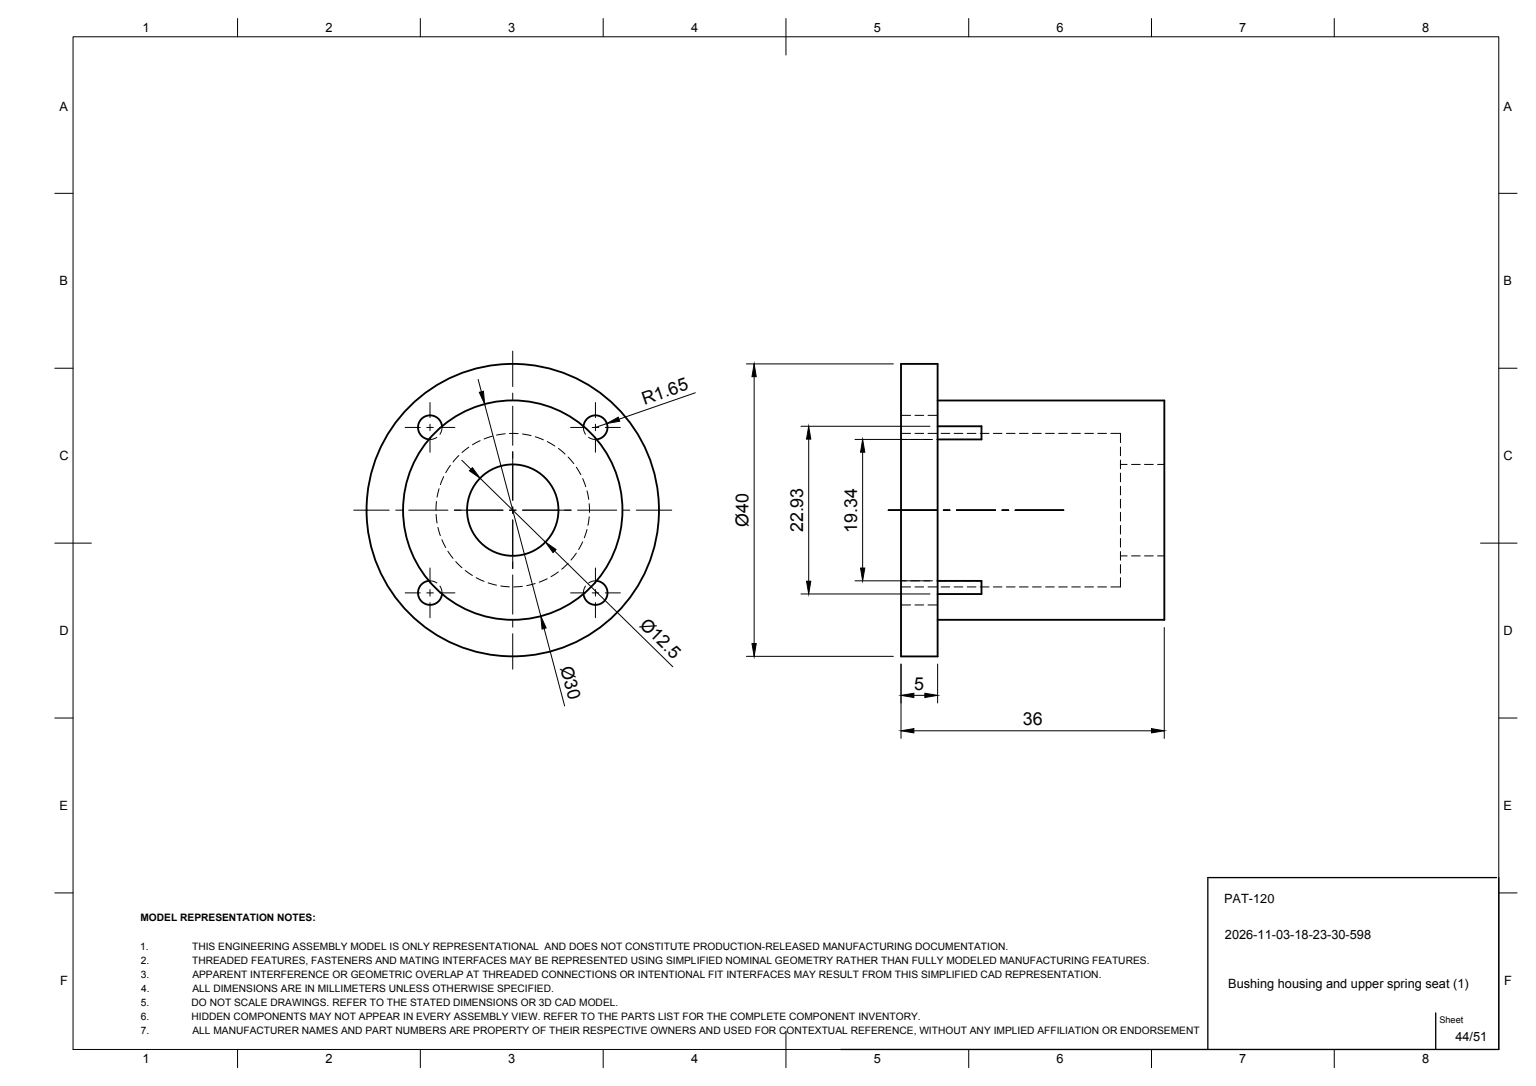
ISO-10303-21;
HEADER;
/* Generated by software containing ST-Developer
 * from STEP Tools, Inc. (www.steptools.com) 
 */

FILE_DESCRIPTION(
/* description */ ('Vibration shaker table dummy'),
/* implementation_level */ '2;1');

FILE_NAME(
/* name */ 'Bushing housing and upper spring seat (1).step',
/* time_stamp */ '2026-10-27T10:55:14-07:00',
/* author */ (''),
/* organization */ (''),
/* preprocessor_version */ 'ST-DEVELOPER v20.2',
/* originating_system */ 'Autodesk Translation Framework v15.17.0.0',
/* authorisation */ '');

FILE_SCHEMA (('AUTOMOTIVE_DESIGN { 1 0 10303 214 3 1 1 }'));
ENDSEC;

DATA;
#10=MECHANICAL_DESIGN_GEOMETRIC_PRESENTATION_REPRESENTATION('',(#725),#22394);
#633=SHAPE_REPRESENTATION_RELATIONSHIP('SRR','None',#22680,#679);
#679=ADVANCED_BREP_SHAPE_REPRESENTATION('',(#769),#22386);
#725=STYLED_ITEM('',(#22961),#769);
#769=MANIFOLD_SOLID_BREP('Body1',#9245);
#1015=FACE_BOUND('',#2489,.T.);
#1016=FACE_BOUND('',#2491,.T.);
#1017=FACE_BOUND('',#2495,.T.);
#1018=FACE_BOUND('',#2496,.T.);
#1019=FACE_BOUND('',#2497,.T.);
#1020=FACE_BOUND('',#2498,.T.);
#1021=FACE_BOUND('',#2499,.T.);
#1022=FACE_BOUND('',#2501,.T.);
#1286=PLANE('',#10567);
#1287=PLANE('',#10574);
#1288=PLANE('',#10581);
#1289=PLANE('',#10588);
#1290=PLANE('',#10605);
#1291=PLANE('',#10607);
#1292=PLANE('',#10613);
#1293=PLANE('',#10614);
#1740=FACE_OUTER_BOUND('',#2478,.T.);
#1741=FACE_OUTER_BOUND('',#2479,.T.);
#1742=FACE_OUTER_BOUND('',#2480,.T.);
#1743=FACE_OUTER_BOUND('',#2481,.T.);
#1744=FACE_OUTER_BOUND('',#2482,.T.);
#1745=FACE_OUTER_BOUND('',#2483,.T.);
#1746=FACE_OUTER_BOUND('',#2484,.T.);
#1747=FACE_OUTER_BOUND('',#2485,.T.);
#1748=FACE_OUTER_BOUND('',#2486,.T.);
#1749=FACE_OUTER_BOUND('',#2487,.T.);
#1750=FACE_OUTER_BOUND('',#2488,.T.);
#1751=FACE_OUTER_BOUND('',#2490,.T.);
#1752=FACE_OUTER_BOUND('',#2492,.T.);
#1753=FACE_OUTER_BOUND('',#2493,.T.);
#1754=FACE_OUTER_BOUND('',#2494,.T.);
#1755=FACE_OUTER_BOUND('',#2500,.T.);
#2478=EDGE_LOOP('',(#8022,#8023));
#2479=EDGE_LOOP('',(#8024,#8025,#8026,#8027,#8028,#8029,#8030,#8031));
#2480=EDGE_LOOP('',(#8032,#8033));
#2481=EDGE_LOOP('',(#8034,#8035,#8036,#8037,#8038,#8039,#8040,#8041));
#2482=EDGE_LOOP('',(#8042,#8043,#8044));
#2483=EDGE_LOOP('',(#8045,#8046,#8047,#8048,#8049,#8050,#8051,#8052));
#2484=EDGE_LOOP('',(#8053,#8054,#8055));
#2485=EDGE_LOOP('',(#8056,#8057,#8058,#8059,#8060,#8061,#8062,#8063));
#2486=EDGE_LOOP('',(#8064,#8065,#8066,#8067,#8068,#8069,#8070,#8071,#8072,
#8073,#8074,#8075,#8076,#8077,#8078,#8079,#8080,#8081,#8082,#8083));
#2487=EDGE_LOOP('',(#8084,#8085,#8086,#8087));
#2488=EDGE_LOOP('',(#8088));
#2489=EDGE_LOOP('',(#8089));
#2490=EDGE_LOOP('',(#8090));
#2491=EDGE_LOOP('',(#8091,#8092,#8093,#8094,#8095,#8096,#8097,#8098,#8099,
#8100,#8101));
#2492=EDGE_LOOP('',(#8102,#8103,#8104,#8105));
#2493=EDGE_LOOP('',(#8106,#8107,#8108,#8109));
#2494=EDGE_LOOP('',(#8110));
#2495=EDGE_LOOP('',(#8111));
#2496=EDGE_LOOP('',(#8112));
#2497=EDGE_LOOP('',(#8113));
#2498=EDGE_LOOP('',(#8114));
#2499=EDGE_LOOP('',(#8115));
#2500=EDGE_LOOP('',(#8116));
#2501=EDGE_LOOP('',(#8117));
#3137=LINE('',#21653,#3756);
#3138=LINE('',#21657,#3757);
#3139=LINE('',#21661,#3758);
#3140=LINE('',#21669,#3759);
#3141=LINE('',#21673,#3760);
#3142=LINE('',#21677,#3761);
#3143=LINE('',#21687,#3762);
#3144=LINE('',#21690,#3763);
#3145=LINE('',#21692,#3764);
#3146=LINE('',#21703,#3765);
#3147=LINE('',#21706,#3766);
#3148=LINE('',#21708,#3767);
#3149=LINE('',#21714,#3768);
#3150=LINE('',#21724,#3769);
#3151=LINE('',#21735,#3770);
#3152=LINE('',#21738,#3771);
#3756=VECTOR('',#13087,1.);
#3757=VECTOR('',#13090,0.165);
#3758=VECTOR('',#13095,1.);
#3759=VECTOR('',#13104,1.);
#3760=VECTOR('',#13107,0.165);
#3761=VECTOR('',#13112,1.);
#3762=VECTOR('',#13123,1.);
#3763=VECTOR('',#13126,1.);
#3764=VECTOR('',#13127,0.165);
#3765=VECTOR('',#13140,1.);
#3766=VECTOR('',#13143,1.);
#3767=VECTOR('',#13144,0.165);
#3768=VECTOR('',#13151,1.5);
#3769=VECTOR('',#13166,1.05);
#3770=VECTOR('',#13181,2.);
#3771=VECTOR('',#13184,0.625);
#4229=CIRCLE('',#10568,1.5);
#4230=CIRCLE('',#10569,0.165);
#4231=CIRCLE('',#10571,0.165);
#4232=CIRCLE('',#10572,0.165);
#4233=CIRCLE('',#10573,0.165);
#4234=CIRCLE('',#10575,1.5);
#4235=CIRCLE('',#10576,0.165);
#4236=CIRCLE('',#10578,0.165);
#4237=CIRCLE('',#10579,0.165);
#4238=CIRCLE('',#10580,0.165);
#4239=CIRCLE('',#10582,1.5);
#4240=CIRCLE('',#10583,0.165);
#4241=CIRCLE('',#10584,0.165);
#4242=CIRCLE('',#10586,0.165);
#4243=CIRCLE('',#10587,0.165);
#4244=CIRCLE('',#10589,1.5);
#4245=CIRCLE('',#10590,0.165);
#4246=CIRCLE('',#10591,0.165);
#4247=CIRCLE('',#10593,0.165);
#4248=CIRCLE('',#10594,0.165);
#4249=CIRCLE('',#10596,1.5);
#4250=CIRCLE('',#10597,1.5);
#4251=CIRCLE('',#10598,1.5);
#4252=CIRCLE('',#10599,1.5);
#4253=CIRCLE('',#10600,1.5);
#4254=CIRCLE('',#10601,1.5);
#4255=CIRCLE('',#10603,1.05);
#4256=CIRCLE('',#10604,1.05);
#4257=CIRCLE('',#10606,0.625);
#4258=CIRCLE('',#10608,2.);
#4259=CIRCLE('',#10610,2.);
#4260=CIRCLE('',#10612,0.625);
#4956=VERTEX_POINT('',#21647);
#4957=VERTEX_POINT('',#21648);
#4958=VERTEX_POINT('',#21652);
#4959=VERTEX_POINT('',#21654);
#4960=VERTEX_POINT('',#21656);
#4961=VERTEX_POINT('',#21659);
#4962=VERTEX_POINT('',#21663);
#4963=VERTEX_POINT('',#21664);
#4964=VERTEX_POINT('',#21668);
#4965=VERTEX_POINT('',#21670);
#4966=VERTEX_POINT('',#21672);
#4967=VERTEX_POINT('',#21675);
#4968=VERTEX_POINT('',#21679);
#4969=VERTEX_POINT('',#21680);
#4970=VERTEX_POINT('',#21682);
#4971=VERTEX_POINT('',#21686);
#4972=VERTEX_POINT('',#21688);
#4973=VERTEX_POINT('',#21691);
#4974=VERTEX_POINT('',#21695);
#4975=VERTEX_POINT('',#21696);
#4976=VERTEX_POINT('',#21698);
#4977=VERTEX_POINT('',#21702);
#4978=VERTEX_POINT('',#21704);
#4979=VERTEX_POINT('',#21707);
#4980=VERTEX_POINT('',#21711);
#4981=VERTEX_POINT('',#21713);
#4982=VERTEX_POINT('',#21721);
#4983=VERTEX_POINT('',#21723);
#4984=VERTEX_POINT('',#21727);
#4985=VERTEX_POINT('',#21730);
#4986=VERTEX_POINT('',#21733);
#4987=VERTEX_POINT('',#21737);
#6004=EDGE_CURVE('',#4956,#4957,#4229,.T.);
#6005=EDGE_CURVE('',#4956,#4957,#4230,.T.);
#6006=EDGE_CURVE('',#4958,#4956,#3137,.T.);
#6007=EDGE_CURVE('',#4959,#4958,#4231,.T.);
#6008=EDGE_CURVE('',#4959,#4960,#3138,.T.);
#6009=EDGE_CURVE('',#4960,#4960,#4232,.T.);
#6010=EDGE_CURVE('',#4961,#4959,#4233,.T.);
#6011=EDGE_CURVE('',#4957,#4961,#3139,.T.);
#6012=EDGE_CURVE('',#4962,#4963,#4234,.T.);
#6013=EDGE_CURVE('',#4962,#4963,#4235,.T.);
#6014=EDGE_CURVE('',#4964,#4962,#3140,.T.);
#6015=EDGE_CURVE('',#4965,#4964,#4236,.T.);
#6016=EDGE_CURVE('',#4965,#4966,#3141,.T.);
#6017=EDGE_CURVE('',#4966,#4966,#4237,.T.);
#6018=EDGE_CURVE('',#4967,#4965,#4238,.T.);
#6019=EDGE_CURVE('',#4963,#4967,#3142,.T.);
#6020=EDGE_CURVE('',#4968,#4969,#4239,.T.);
#6021=EDGE_CURVE('',#4968,#4970,#4240,.T.);
#6022=EDGE_CURVE('',#4970,#4969,#4241,.T.);
#6023=EDGE_CURVE('',#4971,#4968,#3143,.T.);
#6024=EDGE_CURVE('',#4972,#4971,#4242,.T.);
#6025=EDGE_CURVE('',#4969,#4972,#3144,.T.);
#6026=EDGE_CURVE('',#4970,#4973,#3145,.T.);
#6027=EDGE_CURVE('',#4973,#4973,#4243,.T.);
#6028=EDGE_CURVE('',#4974,#4975,#4244,.T.);
#6029=EDGE_CURVE('',#4974,#4976,#4245,.T.);
#6030=EDGE_CURVE('',#4976,#4975,#4246,.T.);
#6031=EDGE_CURVE('',#4977,#4974,#3146,.T.);
#6032=EDGE_CURVE('',#4978,#4977,#4247,.T.);
#6033=EDGE_CURVE('',#4975,#4978,#3147,.T.);
#6034=EDGE_CURVE('',#4976,#4979,#3148,.T.);
#6035=EDGE_CURVE('',#4979,#4979,#4248,.T.);
#6036=EDGE_CURVE('',#4961,#4980,#4249,.T.);
#6037=EDGE_CURVE('',#4980,#4981,#3149,.T.);
#6038=EDGE_CURVE('',#4981,#4981,#4250,.T.);
#6039=EDGE_CURVE('',#4980,#4964,#4251,.T.);
#6040=EDGE_CURVE('',#4967,#4971,#4252,.T.);
#6041=EDGE_CURVE('',#4972,#4977,#4253,.T.);
#6042=EDGE_CURVE('',#4978,#4958,#4254,.T.);
#6043=EDGE_CURVE('',#4982,#4982,#4255,.T.);
#6044=EDGE_CURVE('',#4982,#4983,#3150,.T.);
#6045=EDGE_CURVE('',#4983,#4983,#4256,.T.);
#6046=EDGE_CURVE('',#4984,#4984,#4257,.T.);
#6047=EDGE_CURVE('',#4985,#4985,#4258,.T.);
#6048=EDGE_CURVE('',#4986,#4986,#4259,.T.);
#6049=EDGE_CURVE('',#4986,#4985,#3151,.T.);
#6050=EDGE_CURVE('',#4984,#4987,#3152,.T.);
#6051=EDGE_CURVE('',#4987,#4987,#4260,.T.);
#8022=ORIENTED_EDGE('',*,*,#6004,.F.);
#8023=ORIENTED_EDGE('',*,*,#6005,.T.);
#8024=ORIENTED_EDGE('',*,*,#6006,.F.);
#8025=ORIENTED_EDGE('',*,*,#6007,.F.);
#8026=ORIENTED_EDGE('',*,*,#6008,.T.);
#8027=ORIENTED_EDGE('',*,*,#6009,.F.);
#8028=ORIENTED_EDGE('',*,*,#6008,.F.);
#8029=ORIENTED_EDGE('',*,*,#6010,.F.);
#8030=ORIENTED_EDGE('',*,*,#6011,.F.);
#8031=ORIENTED_EDGE('',*,*,#6005,.F.);
#8032=ORIENTED_EDGE('',*,*,#6012,.F.);
#8033=ORIENTED_EDGE('',*,*,#6013,.T.);
#8034=ORIENTED_EDGE('',*,*,#6014,.F.);
#8035=ORIENTED_EDGE('',*,*,#6015,.F.);
#8036=ORIENTED_EDGE('',*,*,#6016,.T.);
#8037=ORIENTED_EDGE('',*,*,#6017,.F.);
#8038=ORIENTED_EDGE('',*,*,#6016,.F.);
#8039=ORIENTED_EDGE('',*,*,#6018,.F.);
#8040=ORIENTED_EDGE('',*,*,#6019,.F.);
#8041=ORIENTED_EDGE('',*,*,#6013,.F.);
#8042=ORIENTED_EDGE('',*,*,#6020,.F.);
#8043=ORIENTED_EDGE('',*,*,#6021,.T.);
#8044=ORIENTED_EDGE('',*,*,#6022,.T.);
#8045=ORIENTED_EDGE('',*,*,#6023,.F.);
#8046=ORIENTED_EDGE('',*,*,#6024,.F.);
#8047=ORIENTED_EDGE('',*,*,#6025,.F.);
#8048=ORIENTED_EDGE('',*,*,#6022,.F.);
#8049=ORIENTED_EDGE('',*,*,#6026,.T.);
#8050=ORIENTED_EDGE('',*,*,#6027,.F.);
#8051=ORIENTED_EDGE('',*,*,#6026,.F.);
#8052=ORIENTED_EDGE('',*,*,#6021,.F.);
#8053=ORIENTED_EDGE('',*,*,#6028,.F.);
#8054=ORIENTED_EDGE('',*,*,#6029,.T.);
#8055=ORIENTED_EDGE('',*,*,#6030,.T.);
#8056=ORIENTED_EDGE('',*,*,#6031,.F.);
#8057=ORIENTED_EDGE('',*,*,#6032,.F.);
#8058=ORIENTED_EDGE('',*,*,#6033,.F.);
#8059=ORIENTED_EDGE('',*,*,#6030,.F.);
#8060=ORIENTED_EDGE('',*,*,#6034,.T.);
#8061=ORIENTED_EDGE('',*,*,#6035,.F.);
#8062=ORIENTED_EDGE('',*,*,#6034,.F.);
#8063=ORIENTED_EDGE('',*,*,#6029,.F.);
#8064=ORIENTED_EDGE('',*,*,#6006,.T.);
#8065=ORIENTED_EDGE('',*,*,#6004,.T.);
#8066=ORIENTED_EDGE('',*,*,#6011,.T.);
#8067=ORIENTED_EDGE('',*,*,#6036,.T.);
#8068=ORIENTED_EDGE('',*,*,#6037,.T.);
#8069=ORIENTED_EDGE('',*,*,#6038,.T.);
#8070=ORIENTED_EDGE('',*,*,#6037,.F.);
#8071=ORIENTED_EDGE('',*,*,#6039,.T.);
#8072=ORIENTED_EDGE('',*,*,#6014,.T.);
#8073=ORIENTED_EDGE('',*,*,#6012,.T.);
#8074=ORIENTED_EDGE('',*,*,#6019,.T.);
#8075=ORIENTED_EDGE('',*,*,#6040,.T.);
#8076=ORIENTED_EDGE('',*,*,#6023,.T.);
#8077=ORIENTED_EDGE('',*,*,#6020,.T.);
#8078=ORIENTED_EDGE('',*,*,#6025,.T.);
#8079=ORIENTED_EDGE('',*,*,#6041,.T.);
#8080=ORIENTED_EDGE('',*,*,#6031,.T.);
#8081=ORIENTED_EDGE('',*,*,#6028,.T.);
#8082=ORIENTED_EDGE('',*,*,#6033,.T.);
#8083=ORIENTED_EDGE('',*,*,#6042,.T.);
#8084=ORIENTED_EDGE('',*,*,#6043,.F.);
#8085=ORIENTED_EDGE('',*,*,#6044,.T.);
#8086=ORIENTED_EDGE('',*,*,#6045,.F.);
#8087=ORIENTED_EDGE('',*,*,#6044,.F.);
#8088=ORIENTED_EDGE('',*,*,#6043,.T.);
#8089=ORIENTED_EDGE('',*,*,#6046,.F.);
#8090=ORIENTED_EDGE('',*,*,#6047,.F.);
#8091=ORIENTED_EDGE('',*,*,#6010,.T.);
#8092=ORIENTED_EDGE('',*,*,#6007,.T.);
#8093=ORIENTED_EDGE('',*,*,#6042,.F.);
#8094=ORIENTED_EDGE('',*,*,#6032,.T.);
#8095=ORIENTED_EDGE('',*,*,#6041,.F.);
#8096=ORIENTED_EDGE('',*,*,#6024,.T.);
#8097=ORIENTED_EDGE('',*,*,#6040,.F.);
#8098=ORIENTED_EDGE('',*,*,#6018,.T.);
#8099=ORIENTED_EDGE('',*,*,#6015,.T.);
#8100=ORIENTED_EDGE('',*,*,#6039,.F.);
#8101=ORIENTED_EDGE('',*,*,#6036,.F.);
#8102=ORIENTED_EDGE('',*,*,#6048,.F.);
#8103=ORIENTED_EDGE('',*,*,#6049,.T.);
#8104=ORIENTED_EDGE('',*,*,#6047,.T.);
#8105=ORIENTED_EDGE('',*,*,#6049,.F.);
#8106=ORIENTED_EDGE('',*,*,#6046,.T.);
#8107=ORIENTED_EDGE('',*,*,#6050,.T.);
#8108=ORIENTED_EDGE('',*,*,#6051,.T.);
#8109=ORIENTED_EDGE('',*,*,#6050,.F.);
#8110=ORIENTED_EDGE('',*,*,#6048,.T.);
#8111=ORIENTED_EDGE('',*,*,#6045,.T.);
#8112=ORIENTED_EDGE('',*,*,#6035,.T.);
#8113=ORIENTED_EDGE('',*,*,#6027,.T.);
#8114=ORIENTED_EDGE('',*,*,#6017,.T.);
#8115=ORIENTED_EDGE('',*,*,#6009,.T.);
#8116=ORIENTED_EDGE('',*,*,#6038,.F.);
#8117=ORIENTED_EDGE('',*,*,#6051,.F.);
#8666=CYLINDRICAL_SURFACE('',#10570,0.165);
#8667=CYLINDRICAL_SURFACE('',#10577,0.165);
#8668=CYLINDRICAL_SURFACE('',#10585,0.165);
#8669=CYLINDRICAL_SURFACE('',#10592,0.165);
#8670=CYLINDRICAL_SURFACE('',#10595,1.5);
#8671=CYLINDRICAL_SURFACE('',#10602,1.05);
#8672=CYLINDRICAL_SURFACE('',#10609,2.);
#8673=CYLINDRICAL_SURFACE('',#10611,0.625);
#9105=ADVANCED_FACE('',(#1740),#1286,.T.);
#9106=ADVANCED_FACE('',(#1741),#8666,.F.);
#9107=ADVANCED_FACE('',(#1742),#1287,.T.);
#9108=ADVANCED_FACE('',(#1743),#8667,.F.);
#9109=ADVANCED_FACE('',(#1744),#1288,.T.);
#9110=ADVANCED_FACE('',(#1745),#8668,.F.);
#9111=ADVANCED_FACE('',(#1746),#1289,.T.);
#9112=ADVANCED_FACE('',(#1747),#8669,.F.);
#9113=ADVANCED_FACE('',(#1748),#8670,.T.);
#9114=ADVANCED_FACE('',(#1749),#8671,.F.);
#9115=ADVANCED_FACE('',(#1750,#1015),#1290,.T.);
#9116=ADVANCED_FACE('',(#1751,#1016),#1291,.F.);
#9117=ADVANCED_FACE('',(#1752),#8672,.T.);
#9118=ADVANCED_FACE('',(#1753),#8673,.F.);
#9119=ADVANCED_FACE('',(#1754,#1017,#1018,#1019,#1020,#1021),#1292,.T.);
#9120=ADVANCED_FACE('',(#1755,#1022),#1293,.F.);
#9245=CLOSED_SHELL('',(#9105,#9106,#9107,#9108,#9109,#9110,#9111,#9112,
#9113,#9114,#9115,#9116,#9117,#9118,#9119,#9120));
#10566=AXIS2_PLACEMENT_3D('',#21645,#13077,#13078);
#10567=AXIS2_PLACEMENT_3D('',#21646,#13079,#13080);
#10568=AXIS2_PLACEMENT_3D('',#21649,#13081,#13082);
#10569=AXIS2_PLACEMENT_3D('',#21650,#13083,#13084);
#10570=AXIS2_PLACEMENT_3D('',#21651,#13085,#13086);
#10571=AXIS2_PLACEMENT_3D('',#21655,#13088,#13089);
#10572=AXIS2_PLACEMENT_3D('',#21658,#13091,#13092);
#10573=AXIS2_PLACEMENT_3D('',#21660,#13093,#13094);
#10574=AXIS2_PLACEMENT_3D('',#21662,#13096,#13097);
#10575=AXIS2_PLACEMENT_3D('',#21665,#13098,#13099);
#10576=AXIS2_PLACEMENT_3D('',#21666,#13100,#13101);
#10577=AXIS2_PLACEMENT_3D('',#21667,#13102,#13103);
#10578=AXIS2_PLACEMENT_3D('',#21671,#13105,#13106);
#10579=AXIS2_PLACEMENT_3D('',#21674,#13108,#13109);
#10580=AXIS2_PLACEMENT_3D('',#21676,#13110,#13111);
#10581=AXIS2_PLACEMENT_3D('',#21678,#13113,#13114);
#10582=AXIS2_PLACEMENT_3D('',#21681,#13115,#13116);
#10583=AXIS2_PLACEMENT_3D('',#21683,#13117,#13118);
#10584=AXIS2_PLACEMENT_3D('',#21684,#13119,#13120);
#10585=AXIS2_PLACEMENT_3D('',#21685,#13121,#13122);
#10586=AXIS2_PLACEMENT_3D('',#21689,#13124,#13125);
#10587=AXIS2_PLACEMENT_3D('',#21693,#13128,#13129);
#10588=AXIS2_PLACEMENT_3D('',#21694,#13130,#13131);
#10589=AXIS2_PLACEMENT_3D('',#21697,#13132,#13133);
#10590=AXIS2_PLACEMENT_3D('',#21699,#13134,#13135);
#10591=AXIS2_PLACEMENT_3D('',#21700,#13136,#13137);
#10592=AXIS2_PLACEMENT_3D('',#21701,#13138,#13139);
#10593=AXIS2_PLACEMENT_3D('',#21705,#13141,#13142);
#10594=AXIS2_PLACEMENT_3D('',#21709,#13145,#13146);
#10595=AXIS2_PLACEMENT_3D('',#21710,#13147,#13148);
#10596=AXIS2_PLACEMENT_3D('',#21712,#13149,#13150);
#10597=AXIS2_PLACEMENT_3D('',#21715,#13152,#13153);
#10598=AXIS2_PLACEMENT_3D('',#21716,#13154,#13155);
#10599=AXIS2_PLACEMENT_3D('',#21717,#13156,#13157);
#10600=AXIS2_PLACEMENT_3D('',#21718,#13158,#13159);
#10601=AXIS2_PLACEMENT_3D('',#21719,#13160,#13161);
#10602=AXIS2_PLACEMENT_3D('',#21720,#13162,#13163);
#10603=AXIS2_PLACEMENT_3D('',#21722,#13164,#13165);
#10604=AXIS2_PLACEMENT_3D('',#21725,#13167,#13168);
#10605=AXIS2_PLACEMENT_3D('',#21726,#13169,#13170);
#10606=AXIS2_PLACEMENT_3D('',#21728,#13171,#13172);
#10607=AXIS2_PLACEMENT_3D('',#21729,#13173,#13174);
#10608=AXIS2_PLACEMENT_3D('',#21731,#13175,#13176);
#10609=AXIS2_PLACEMENT_3D('',#21732,#13177,#13178);
#10610=AXIS2_PLACEMENT_3D('',#21734,#13179,#13180);
#10611=AXIS2_PLACEMENT_3D('',#21736,#13182,#13183);
#10612=AXIS2_PLACEMENT_3D('',#21739,#13185,#13186);
#10613=AXIS2_PLACEMENT_3D('',#21740,#13187,#13188);
#10614=AXIS2_PLACEMENT_3D('',#21741,#13189,#13190);
#13077=DIRECTION('axis',(0.,0.,1.));
#13078=DIRECTION('refdir',(1.,0.,0.));
#13079=DIRECTION('center_axis',(0.,0.,1.));
#13080=DIRECTION('ref_axis',(1.,0.,0.));
#13081=DIRECTION('center_axis',(0.,0.,-1.));
#13082=DIRECTION('ref_axis',(1.,0.,0.));
#13083=DIRECTION('center_axis',(0.,0.,1.));
#13084=DIRECTION('ref_axis',(1.,0.,0.));
#13085=DIRECTION('center_axis',(0.,0.,1.));
#13086=DIRECTION('ref_axis',(1.,0.,0.));
#13087=DIRECTION('',(0.,0.,-1.));
#13088=DIRECTION('center_axis',(0.,0.,1.));
#13089=DIRECTION('ref_axis',(1.,0.,0.));
#13090=DIRECTION('',(0.,0.,1.));
#13091=DIRECTION('center_axis',(0.,0.,-1.));
#13092=DIRECTION('ref_axis',(1.,0.,0.));
#13093=DIRECTION('center_axis',(0.,0.,1.));
#13094=DIRECTION('ref_axis',(1.,0.,0.));
#13095=DIRECTION('',(0.,0.,1.));
#13096=DIRECTION('center_axis',(0.,0.,1.));
#13097=DIRECTION('ref_axis',(1.,0.,0.));
#13098=DIRECTION('center_axis',(0.,0.,-1.));
#13099=DIRECTION('ref_axis',(1.,0.,0.));
#13100=DIRECTION('center_axis',(0.,0.,1.));
#13101=DIRECTION('ref_axis',(1.,0.,0.));
#13102=DIRECTION('center_axis',(0.,0.,1.));
#13103=DIRECTION('ref_axis',(1.,0.,0.));
#13104=DIRECTION('',(0.,0.,-1.));
#13105=DIRECTION('center_axis',(0.,0.,1.));
#13106=DIRECTION('ref_axis',(1.,0.,0.));
#13107=DIRECTION('',(0.,0.,1.));
#13108=DIRECTION('center_axis',(0.,0.,-1.));
#13109=DIRECTION('ref_axis',(1.,0.,0.));
#13110=DIRECTION('center_axis',(0.,0.,1.));
#13111=DIRECTION('ref_axis',(1.,0.,0.));
#13112=DIRECTION('',(0.,0.,1.));
#13113=DIRECTION('center_axis',(0.,0.,1.));
#13114=DIRECTION('ref_axis',(1.,0.,0.));
#13115=DIRECTION('center_axis',(0.,0.,-1.));
#13116=DIRECTION('ref_axis',(1.,0.,0.));
#13117=DIRECTION('center_axis',(0.,0.,1.));
#13118=DIRECTION('ref_axis',(1.,0.,0.));
#13119=DIRECTION('center_axis',(0.,0.,1.));
#13120=DIRECTION('ref_axis',(1.,0.,0.));
#13121=DIRECTION('center_axis',(0.,0.,1.));
#13122=DIRECTION('ref_axis',(1.,0.,0.));
#13123=DIRECTION('',(0.,0.,-1.));
#13124=DIRECTION('center_axis',(0.,0.,1.));
#13125=DIRECTION('ref_axis',(1.,0.,0.));
#13126=DIRECTION('',(0.,0.,1.));
#13127=DIRECTION('',(0.,0.,1.));
#13128=DIRECTION('center_axis',(0.,0.,-1.));
#13129=DIRECTION('ref_axis',(1.,0.,0.));
#13130=DIRECTION('center_axis',(0.,0.,1.));
#13131=DIRECTION('ref_axis',(1.,0.,0.));
#13132=DIRECTION('center_axis',(0.,0.,-1.));
#13133=DIRECTION('ref_axis',(1.,0.,0.));
#13134=DIRECTION('center_axis',(0.,0.,1.));
#13135=DIRECTION('ref_axis',(1.,0.,0.));
#13136=DIRECTION('center_axis',(0.,0.,1.));
#13137=DIRECTION('ref_axis',(1.,0.,0.));
#13138=DIRECTION('center_axis',(0.,0.,1.));
#13139=DIRECTION('ref_axis',(1.,0.,0.));
#13140=DIRECTION('',(0.,0.,-1.));
#13141=DIRECTION('center_axis',(0.,0.,1.));
#13142=DIRECTION('ref_axis',(1.,0.,0.));
#13143=DIRECTION('',(0.,0.,1.));
#13144=DIRECTION('',(0.,0.,1.));
#13145=DIRECTION('center_axis',(0.,0.,-1.));
#13146=DIRECTION('ref_axis',(1.,0.,0.));
#13147=DIRECTION('center_axis',(0.,0.,1.));
#13148=DIRECTION('ref_axis',(1.,0.,0.));
#13149=DIRECTION('center_axis',(0.,0.,-1.));
#13150=DIRECTION('ref_axis',(1.,0.,0.));
#13151=DIRECTION('',(0.,0.,-1.));
#13152=DIRECTION('center_axis',(0.,0.,1.));
#13153=DIRECTION('ref_axis',(1.,0.,0.));
#13154=DIRECTION('center_axis',(0.,0.,-1.));
#13155=DIRECTION('ref_axis',(1.,0.,0.));
#13156=DIRECTION('center_axis',(0.,0.,-1.));
#13157=DIRECTION('ref_axis',(1.,0.,0.));
#13158=DIRECTION('center_axis',(0.,0.,-1.));
#13159=DIRECTION('ref_axis',(1.,0.,0.));
#13160=DIRECTION('center_axis',(0.,0.,-1.));
#13161=DIRECTION('ref_axis',(1.,0.,0.));
#13162=DIRECTION('center_axis',(0.,0.,1.));
#13163=DIRECTION('ref_axis',(1.,0.,0.));
#13164=DIRECTION('center_axis',(0.,0.,1.));
#13165=DIRECTION('ref_axis',(1.,0.,0.));
#13166=DIRECTION('',(0.,0.,1.));
#13167=DIRECTION('center_axis',(0.,0.,-1.));
#13168=DIRECTION('ref_axis',(1.,0.,0.));
#13169=DIRECTION('center_axis',(0.,0.,1.));
#13170=DIRECTION('ref_axis',(1.,0.,0.));
#13171=DIRECTION('center_axis',(0.,0.,1.));
#13172=DIRECTION('ref_axis',(1.,0.,0.));
#13173=DIRECTION('center_axis',(0.,0.,1.));
#13174=DIRECTION('ref_axis',(1.,0.,0.));
#13175=DIRECTION('center_axis',(0.,0.,1.));
#13176=DIRECTION('ref_axis',(1.,0.,0.));
#13177=DIRECTION('center_axis',(0.,0.,1.));
#13178=DIRECTION('ref_axis',(1.,0.,0.));
#13179=DIRECTION('center_axis',(0.,0.,1.));
#13180=DIRECTION('ref_axis',(1.,0.,0.));
#13181=DIRECTION('',(0.,0.,-1.));
#13182=DIRECTION('center_axis',(0.,0.,1.));
#13183=DIRECTION('ref_axis',(1.,0.,0.));
#13184=DIRECTION('',(0.,0.,-1.));
#13185=DIRECTION('center_axis',(0.,0.,-1.));
#13186=DIRECTION('ref_axis',(1.,0.,0.));
#13187=DIRECTION('center_axis',(0.,0.,1.));
#13188=DIRECTION('ref_axis',(1.,0.,0.));
#13189=DIRECTION('center_axis',(0.,0.,1.));
#13190=DIRECTION('ref_axis',(1.,0.,0.));
#21645=CARTESIAN_POINT('',(0.,0.,0.));
#21646=CARTESIAN_POINT('Origin',(-7.13137084989848,2.86862915010152,14.));
#21647=CARTESIAN_POINT('',(-6.96707794165985,2.85337004454142,14.));
#21648=CARTESIAN_POINT('',(-7.14662995545858,3.03292205834015,14.));
#21649=CARTESIAN_POINT('Origin',(-6.,4.,14.));
#21650=CARTESIAN_POINT('Origin',(-7.13137084989848,2.86862915010152,14.));
#21651=CARTESIAN_POINT('Origin',(-7.13137084989848,2.86862915010152,14.));
#21652=CARTESIAN_POINT('',(-6.96707794165985,2.85337004454142,14.6));
#21653=CARTESIAN_POINT('',(-6.96707794165985,2.85337004454142,14.));
#21654=CARTESIAN_POINT('',(-7.29637084989848,2.86862915010152,14.6));
#21655=CARTESIAN_POINT('Origin',(-7.13137084989848,2.86862915010152,14.6));
#21656=CARTESIAN_POINT('',(-7.29637084989848,2.86862915010152,15.1));
#21657=CARTESIAN_POINT('',(-7.29637084989848,2.86862915010152,14.));
#21658=CARTESIAN_POINT('Origin',(-7.13137084989848,2.86862915010152,15.1));
#21659=CARTESIAN_POINT('',(-7.14662995545858,3.03292205834015,14.6));
#21660=CARTESIAN_POINT('Origin',(-7.13137084989848,2.86862915010152,14.6));
#21661=CARTESIAN_POINT('',(-7.14662995545858,3.03292205834015,14.));
#21662=CARTESIAN_POINT('Origin',(-7.13137084989848,5.13137084989848,14.));
#21663=CARTESIAN_POINT('',(-7.14662995545858,4.96707794165985,14.));
#21664=CARTESIAN_POINT('',(-6.96707794165985,5.14662995545858,14.));
#21665=CARTESIAN_POINT('Origin',(-6.,4.,14.));
#21666=CARTESIAN_POINT('Origin',(-7.13137084989848,5.13137084989848,14.));
#21667=CARTESIAN_POINT('Origin',(-7.13137084989848,5.13137084989848,14.));
#21668=CARTESIAN_POINT('',(-7.14662995545858,4.96707794165985,14.6));
#21669=CARTESIAN_POINT('',(-7.14662995545858,4.96707794165985,14.));
#21670=CARTESIAN_POINT('',(-7.29637084989848,5.13137084989848,14.6));
#21671=CARTESIAN_POINT('Origin',(-7.13137084989848,5.13137084989848,14.6));
#21672=CARTESIAN_POINT('',(-7.29637084989848,5.13137084989848,15.1));
#21673=CARTESIAN_POINT('',(-7.29637084989848,5.13137084989848,14.));
#21674=CARTESIAN_POINT('Origin',(-7.13137084989848,5.13137084989848,15.1));
#21675=CARTESIAN_POINT('',(-6.96707794165985,5.14662995545858,14.6));
#21676=CARTESIAN_POINT('Origin',(-7.13137084989848,5.13137084989848,14.6));
#21677=CARTESIAN_POINT('',(-6.96707794165985,5.14662995545858,14.));
#21678=CARTESIAN_POINT('Origin',(-4.86862915010152,5.13137084989848,14.));
#21679=CARTESIAN_POINT('',(-5.03292205834015,5.14662995545858,14.));
#21680=CARTESIAN_POINT('',(-4.85337004454142,4.96707794165985,14.));
#21681=CARTESIAN_POINT('Origin',(-6.,4.,14.));
#21682=CARTESIAN_POINT('',(-5.03362915010152,5.13137084989848,14.));
#21683=CARTESIAN_POINT('Origin',(-4.86862915010152,5.13137084989848,14.));
#21684=CARTESIAN_POINT('Origin',(-4.86862915010152,5.13137084989848,14.));
#21685=CARTESIAN_POINT('Origin',(-4.86862915010152,5.13137084989848,14.));
#21686=CARTESIAN_POINT('',(-5.03292205834015,5.14662995545858,14.6));
#21687=CARTESIAN_POINT('',(-5.03292205834015,5.14662995545858,14.));
#21688=CARTESIAN_POINT('',(-4.85337004454142,4.96707794165985,14.6));
#21689=CARTESIAN_POINT('Origin',(-4.86862915010152,5.13137084989848,14.6));
#21690=CARTESIAN_POINT('',(-4.85337004454142,4.96707794165985,14.));
#21691=CARTESIAN_POINT('',(-5.03362915010152,5.13137084989848,15.1));
#21692=CARTESIAN_POINT('',(-5.03362915010152,5.13137084989848,14.));
#21693=CARTESIAN_POINT('Origin',(-4.86862915010152,5.13137084989848,15.1));
#21694=CARTESIAN_POINT('Origin',(-4.86862915010152,2.86862915010152,14.));
#21695=CARTESIAN_POINT('',(-4.85337004454142,3.03292205834015,14.));
#21696=CARTESIAN_POINT('',(-5.03292205834015,2.85337004454142,14.));
#21697=CARTESIAN_POINT('Origin',(-6.,4.,14.));
#21698=CARTESIAN_POINT('',(-5.03362915010152,2.86862915010152,14.));
#21699=CARTESIAN_POINT('Origin',(-4.86862915010152,2.86862915010152,14.));
#21700=CARTESIAN_POINT('Origin',(-4.86862915010152,2.86862915010152,14.));
#21701=CARTESIAN_POINT('Origin',(-4.86862915010152,2.86862915010152,14.));
#21702=CARTESIAN_POINT('',(-4.85337004454142,3.03292205834015,14.6));
#21703=CARTESIAN_POINT('',(-4.85337004454142,3.03292205834015,14.));
#21704=CARTESIAN_POINT('',(-5.03292205834015,2.85337004454142,14.6));
#21705=CARTESIAN_POINT('Origin',(-4.86862915010152,2.86862915010152,14.6));
#21706=CARTESIAN_POINT('',(-5.03292205834015,2.85337004454142,14.));
#21707=CARTESIAN_POINT('',(-5.03362915010152,2.86862915010152,15.1));
#21708=CARTESIAN_POINT('',(-5.03362915010152,2.86862915010152,14.));
#21709=CARTESIAN_POINT('Origin',(-4.86862915010152,2.86862915010152,15.1));
#21710=CARTESIAN_POINT('Origin',(-6.,4.,11.5));
#21711=CARTESIAN_POINT('',(-7.5,4.,14.6));
#21712=CARTESIAN_POINT('Origin',(-6.,4.,14.6));
#21713=CARTESIAN_POINT('',(-7.5,4.,11.5));
#21714=CARTESIAN_POINT('',(-7.5,4.,11.5));
#21715=CARTESIAN_POINT('Origin',(-6.,4.,11.5));
#21716=CARTESIAN_POINT('Origin',(-6.,4.,14.6));
#21717=CARTESIAN_POINT('Origin',(-6.,4.,14.6));
#21718=CARTESIAN_POINT('Origin',(-6.,4.,14.6));
#21719=CARTESIAN_POINT('Origin',(-6.,4.,14.6));
#21720=CARTESIAN_POINT('Origin',(-6.,4.,12.1));
#21721=CARTESIAN_POINT('',(-7.05,4.,12.1));
#21722=CARTESIAN_POINT('Origin',(-6.,4.,12.1));
#21723=CARTESIAN_POINT('',(-7.05,4.,15.1));
#21724=CARTESIAN_POINT('',(-7.05,4.,12.1));
#21725=CARTESIAN_POINT('Origin',(-6.,4.,15.1));
#21726=CARTESIAN_POINT('Origin',(-6.,4.,12.1));
#21727=CARTESIAN_POINT('',(-6.625,4.,12.1));
#21728=CARTESIAN_POINT('Origin',(-6.,4.,12.1));
#21729=CARTESIAN_POINT('Origin',(-6.,4.,14.6));
#21730=CARTESIAN_POINT('',(-8.,4.,14.6));
#21731=CARTESIAN_POINT('Origin',(-6.,4.,14.6));
#21732=CARTESIAN_POINT('Origin',(-6.,4.,14.6));
#21733=CARTESIAN_POINT('',(-8.,4.,15.1));
#21734=CARTESIAN_POINT('Origin',(-6.,4.,15.1));
#21735=CARTESIAN_POINT('',(-8.,4.,14.6));
#21736=CARTESIAN_POINT('Origin',(-6.,4.,11.5));
#21737=CARTESIAN_POINT('',(-6.625,4.,11.5));
#21738=CARTESIAN_POINT('',(-6.625,4.,11.5));
#21739=CARTESIAN_POINT('Origin',(-6.,4.,11.5));
#21740=CARTESIAN_POINT('Origin',(-6.,4.,15.1));
#21741=CARTESIAN_POINT('Origin',(-6.,4.,11.5));
#22335=UNCERTAINTY_MEASURE_WITH_UNIT(LENGTH_MEASURE(0.001),#22395,
'DISTANCE_ACCURACY_VALUE',
'Maximum model space distance between geometric entities at asserted c
onnectivities');
#22343=UNCERTAINTY_MEASURE_WITH_UNIT(LENGTH_MEASURE(0.001),#22395,
'DISTANCE_ACCURACY_VALUE',
'Maximum model space distance between geometric entities at asserted c
onnectivities');
#22386=(
GEOMETRIC_REPRESENTATION_CONTEXT(3)
GLOBAL_UNCERTAINTY_ASSIGNED_CONTEXT((#22335))
GLOBAL_UNIT_ASSIGNED_CONTEXT((#22395,#22397,#22398))
REPRESENTATION_CONTEXT('','3D')
);
#22394=(
GEOMETRIC_REPRESENTATION_CONTEXT(3)
GLOBAL_UNCERTAINTY_ASSIGNED_CONTEXT((#22343))
GLOBAL_UNIT_ASSIGNED_CONTEXT((#22395,#22397,#22398))
REPRESENTATION_CONTEXT('','3D')
);
#22395=(
LENGTH_UNIT()
NAMED_UNIT(*)
SI_UNIT(.CENTI.,.METRE.)
);
#22397=(
NAMED_UNIT(*)
PLANE_ANGLE_UNIT()
SI_UNIT($,.RADIAN.)
);
#22398=(
NAMED_UNIT(*)
SI_UNIT($,.STERADIAN.)
SOLID_ANGLE_UNIT()
);
#22441=SHAPE_DEFINITION_REPRESENTATION(#22491,#22680);
#22491=PRODUCT_DEFINITION_SHAPE('',$,#22731);
#22680=SHAPE_REPRESENTATION('',(#10566),#22386);
#22688=PRODUCT_DEFINITION_CONTEXT('part definition',#22840,'design');
#22731=PRODUCT_DEFINITION('Bushing housing and upper spring seat (1)',
'Bushing housing and upper spring seat (1)',#22781,#22688);
#22781=PRODUCT_DEFINITION_FORMATION('',$,#22884);
#22840=APPLICATION_CONTEXT(
'Core Data for Automotive Mechanical Design Process');
#22841=PRODUCT_CONTEXT('part definition',#22840,'mechanical');
#22884=PRODUCT('Bushing housing and upper spring seat (1)',
'Bushing housing and upper spring seat (1)',
'Bushing housing and upper spring seat (1)',(#22841));
#22955=COLOUR_RGB('Grey',0.48,0.52,0.57);
#22956=FILL_AREA_STYLE_COLOUR('',#22955);
#22957=FILL_AREA_STYLE('',(#22956));
#22958=SURFACE_STYLE_FILL_AREA(#22957);
#22959=SURFACE_SIDE_STYLE('',(#22958));
#22960=SURFACE_STYLE_USAGE(.BOTH.,#22959);
#22961=PRESENTATION_STYLE_ASSIGNMENT((#22960));
ENDSEC;
END-ISO-10303-21;
